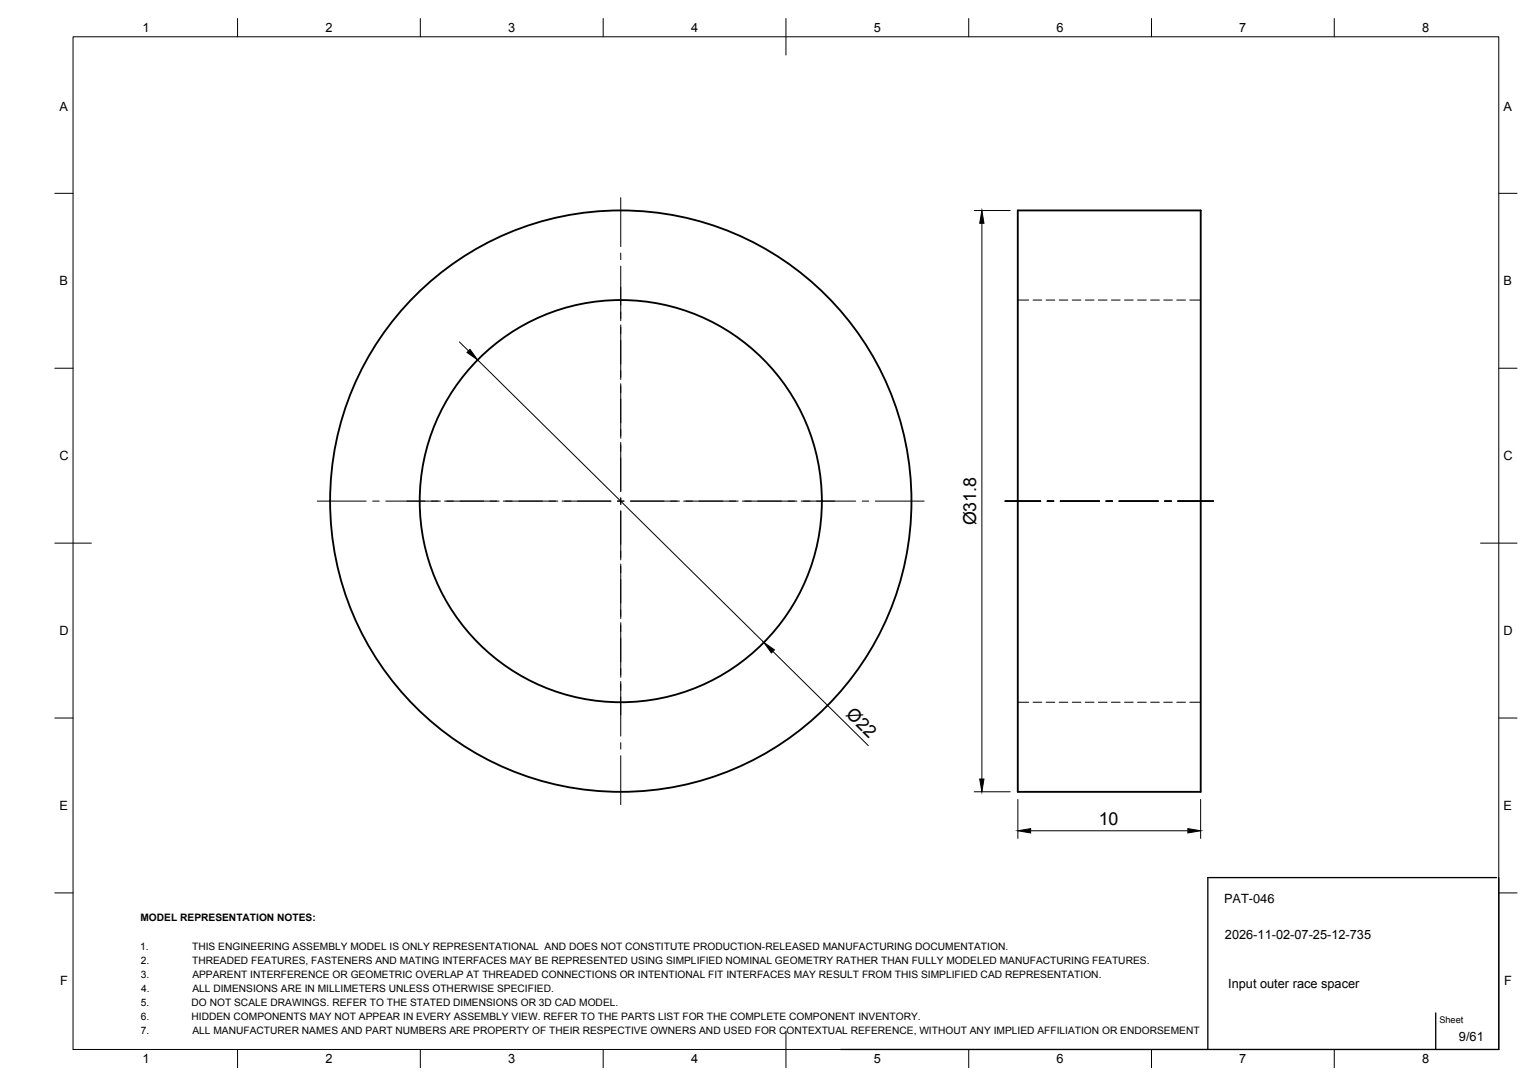
ISO-10303-21;
HEADER;
/* Generated by software containing ST-Developer
 * from STEP Tools, Inc. (www.steptools.com) 
 */

FILE_DESCRIPTION(
/* description */ ('Gear mesh backlash fixture'),
/* implementation_level */ '2;1');

FILE_NAME(
/* name */ 'Input outer race spacer.step',
/* time_stamp */ '2026-10-28T03:26:00-07:00',
/* author */ (''),
/* organization */ (''),
/* preprocessor_version */ 'ST-DEVELOPER v20.2',
/* originating_system */ 'Autodesk Translation Framework v15.17.0.0',
/* authorisation */ '');

FILE_SCHEMA (('AUTOMOTIVE_DESIGN { 1 0 10303 214 3 1 1 }'));
ENDSEC;

DATA;
#10=MECHANICAL_DESIGN_GEOMETRIC_PRESENTATION_REPRESENTATION('',(#1020),#57900);
#920=SHAPE_REPRESENTATION_RELATIONSHIP('SRR','None',#58115,#970);
#970=ADVANCED_BREP_SHAPE_REPRESENTATION('',(#1085),#57848);
#1020=STYLED_ITEM('',(#58465),#1085);
#1085=MANIFOLD_SOLID_BREP('Body1',#13580);
#1185=FACE_BOUND('',#2563,.T.);
#1186=FACE_BOUND('',#2565,.T.);
#1360=PLANE('',#14331);
#1361=PLANE('',#14332);
#1753=FACE_OUTER_BOUND('',#2560,.T.);
#1754=FACE_OUTER_BOUND('',#2561,.T.);
#1755=FACE_OUTER_BOUND('',#2562,.T.);
#1756=FACE_OUTER_BOUND('',#2564,.T.);
#2560=EDGE_LOOP('',(#9153,#9154,#9155,#9156));
#2561=EDGE_LOOP('',(#9157,#9158,#9159,#9160));
#2562=EDGE_LOOP('',(#9161));
#2563=EDGE_LOOP('',(#9162));
#2564=EDGE_LOOP('',(#9163));
#2565=EDGE_LOOP('',(#9164));
#3480=LINE('',#19600,#4369);
#3481=LINE('',#19606,#4370);
#4369=VECTOR('',#15911,1.1);
#4370=VECTOR('',#15918,1.59);
#5253=CIRCLE('',#14326,1.1);
#5254=CIRCLE('',#14327,1.1);
#5255=CIRCLE('',#14329,1.59);
#5256=CIRCLE('',#14330,1.59);
#5873=VERTEX_POINT('',#19597);
#5874=VERTEX_POINT('',#19599);
#5875=VERTEX_POINT('',#19603);
#5876=VERTEX_POINT('',#19605);
#7163=EDGE_CURVE('',#5873,#5873,#5253,.T.);
#7164=EDGE_CURVE('',#5873,#5874,#3480,.T.);
#7165=EDGE_CURVE('',#5874,#5874,#5254,.T.);
#7166=EDGE_CURVE('',#5875,#5875,#5255,.T.);
#7167=EDGE_CURVE('',#5875,#5876,#3481,.T.);
#7168=EDGE_CURVE('',#5876,#5876,#5256,.T.);
#9153=ORIENTED_EDGE('',*,*,#7163,.F.);
#9154=ORIENTED_EDGE('',*,*,#7164,.T.);
#9155=ORIENTED_EDGE('',*,*,#7165,.T.);
#9156=ORIENTED_EDGE('',*,*,#7164,.F.);
#9157=ORIENTED_EDGE('',*,*,#7166,.F.);
#9158=ORIENTED_EDGE('',*,*,#7167,.T.);
#9159=ORIENTED_EDGE('',*,*,#7168,.T.);
#9160=ORIENTED_EDGE('',*,*,#7167,.F.);
#9161=ORIENTED_EDGE('',*,*,#7166,.T.);
#9162=ORIENTED_EDGE('',*,*,#7163,.T.);
#9163=ORIENTED_EDGE('',*,*,#7168,.F.);
#9164=ORIENTED_EDGE('',*,*,#7165,.F.);
#12614=CYLINDRICAL_SURFACE('',#14325,1.1);
#12615=CYLINDRICAL_SURFACE('',#14328,1.59);
#12870=ADVANCED_FACE('',(#1753),#12614,.F.);
#12871=ADVANCED_FACE('',(#1754),#12615,.T.);
#12872=ADVANCED_FACE('',(#1755,#1185),#1360,.T.);
#12873=ADVANCED_FACE('',(#1756,#1186),#1361,.F.);
#13580=CLOSED_SHELL('',(#12870,#12871,#12872,#12873));
#14324=AXIS2_PLACEMENT_3D('',#19595,#15905,#15906);
#14325=AXIS2_PLACEMENT_3D('',#19596,#15907,#15908);
#14326=AXIS2_PLACEMENT_3D('',#19598,#15909,#15910);
#14327=AXIS2_PLACEMENT_3D('',#19601,#15912,#15913);
#14328=AXIS2_PLACEMENT_3D('',#19602,#15914,#15915);
#14329=AXIS2_PLACEMENT_3D('',#19604,#15916,#15917);
#14330=AXIS2_PLACEMENT_3D('',#19607,#15919,#15920);
#14331=AXIS2_PLACEMENT_3D('',#19608,#15921,#15922);
#14332=AXIS2_PLACEMENT_3D('',#19609,#15923,#15924);
#15905=DIRECTION('axis',(0.,0.,1.));
#15906=DIRECTION('refdir',(1.,0.,0.));
#15907=DIRECTION('center_axis',(0.,0.,1.));
#15908=DIRECTION('ref_axis',(1.,0.,0.));
#15909=DIRECTION('center_axis',(0.,0.,-1.));
#15910=DIRECTION('ref_axis',(1.,0.,0.));
#15911=DIRECTION('',(0.,0.,-1.));
#15912=DIRECTION('center_axis',(0.,0.,-1.));
#15913=DIRECTION('ref_axis',(1.,0.,0.));
#15914=DIRECTION('center_axis',(0.,0.,1.));
#15915=DIRECTION('ref_axis',(1.,0.,0.));
#15916=DIRECTION('center_axis',(0.,0.,1.));
#15917=DIRECTION('ref_axis',(1.,0.,0.));
#15918=DIRECTION('',(0.,0.,-1.));
#15919=DIRECTION('center_axis',(0.,0.,1.));
#15920=DIRECTION('ref_axis',(1.,0.,0.));
#15921=DIRECTION('center_axis',(0.,0.,1.));
#15922=DIRECTION('ref_axis',(1.,0.,0.));
#15923=DIRECTION('center_axis',(0.,0.,1.));
#15924=DIRECTION('ref_axis',(1.,0.,0.));
#19595=CARTESIAN_POINT('',(0.,0.,0.));
#19596=CARTESIAN_POINT('Origin',(0.,0.,7.));
#19597=CARTESIAN_POINT('',(-1.1,-1.34711147906209E-16,8.));
#19598=CARTESIAN_POINT('Origin',(0.,0.,8.));
#19599=CARTESIAN_POINT('',(-1.1,-1.34711147906209E-16,7.));
#19600=CARTESIAN_POINT('',(-1.1,-1.34711147906209E-16,7.));
#19601=CARTESIAN_POINT('Origin',(0.,0.,7.));
#19602=CARTESIAN_POINT('Origin',(0.,0.,7.));
#19603=CARTESIAN_POINT('',(-1.59,-1.94718841064429E-16,8.));
#19604=CARTESIAN_POINT('Origin',(0.,0.,8.));
#19605=CARTESIAN_POINT('',(-1.59,-1.94718841064429E-16,7.));
#19606=CARTESIAN_POINT('',(-1.59,-1.94718841064429E-16,7.));
#19607=CARTESIAN_POINT('Origin',(0.,0.,7.));
#19608=CARTESIAN_POINT('Origin',(0.,0.,8.));
#19609=CARTESIAN_POINT('Origin',(0.,0.,7.));
#57789=UNCERTAINTY_MEASURE_WITH_UNIT(LENGTH_MEASURE(0.001),#57901,
'DISTANCE_ACCURACY_VALUE',
'Maximum model space distance between geometric entities at asserted c
onnectivities');
#57841=UNCERTAINTY_MEASURE_WITH_UNIT(LENGTH_MEASURE(0.001),#57901,
'DISTANCE_ACCURACY_VALUE',
'Maximum model space distance between geometric entities at asserted c
onnectivities');
#57848=(
GEOMETRIC_REPRESENTATION_CONTEXT(3)
GLOBAL_UNCERTAINTY_ASSIGNED_CONTEXT((#57789))
GLOBAL_UNIT_ASSIGNED_CONTEXT((#57901,#57903,#57904))
REPRESENTATION_CONTEXT('','3D')
);
#57900=(
GEOMETRIC_REPRESENTATION_CONTEXT(3)
GLOBAL_UNCERTAINTY_ASSIGNED_CONTEXT((#57841))
GLOBAL_UNIT_ASSIGNED_CONTEXT((#57901,#57903,#57904))
REPRESENTATION_CONTEXT('','3D')
);
#57901=(
LENGTH_UNIT()
NAMED_UNIT(*)
SI_UNIT(.CENTI.,.METRE.)
);
#57903=(
NAMED_UNIT(*)
PLANE_ANGLE_UNIT()
SI_UNIT($,.RADIAN.)
);
#57904=(
NAMED_UNIT(*)
SI_UNIT($,.STERADIAN.)
SOLID_ANGLE_UNIT()
);
#57911=SHAPE_DEFINITION_REPRESENTATION(#57969,#58115);
#57969=PRODUCT_DEFINITION_SHAPE('',$,#58174);
#58115=SHAPE_REPRESENTATION('',(#14324),#57848);
#58167=PRODUCT_DEFINITION_CONTEXT('part definition',#58343,'design');
#58174=PRODUCT_DEFINITION('Input outer race spacer',
'Input outer race spacer',#58232,#58167);
#58232=PRODUCT_DEFINITION_FORMATION('',$,#58351);
#58343=APPLICATION_CONTEXT(
'Core Data for Automotive Mechanical Design Process');
#58344=PRODUCT_CONTEXT('part definition',#58343,'mechanical');
#58351=PRODUCT('Input outer race spacer','Input outer race spacer',
'Input outer race spacer',(#58344));
#58459=COLOUR_RGB('Grey',0.48,0.52,0.57);
#58460=FILL_AREA_STYLE_COLOUR('',#58459);
#58461=FILL_AREA_STYLE('',(#58460));
#58462=SURFACE_STYLE_FILL_AREA(#58461);
#58463=SURFACE_SIDE_STYLE('',(#58462));
#58464=SURFACE_STYLE_USAGE(.BOTH.,#58463);
#58465=PRESENTATION_STYLE_ASSIGNMENT((#58464));
ENDSEC;
END-ISO-10303-21;
